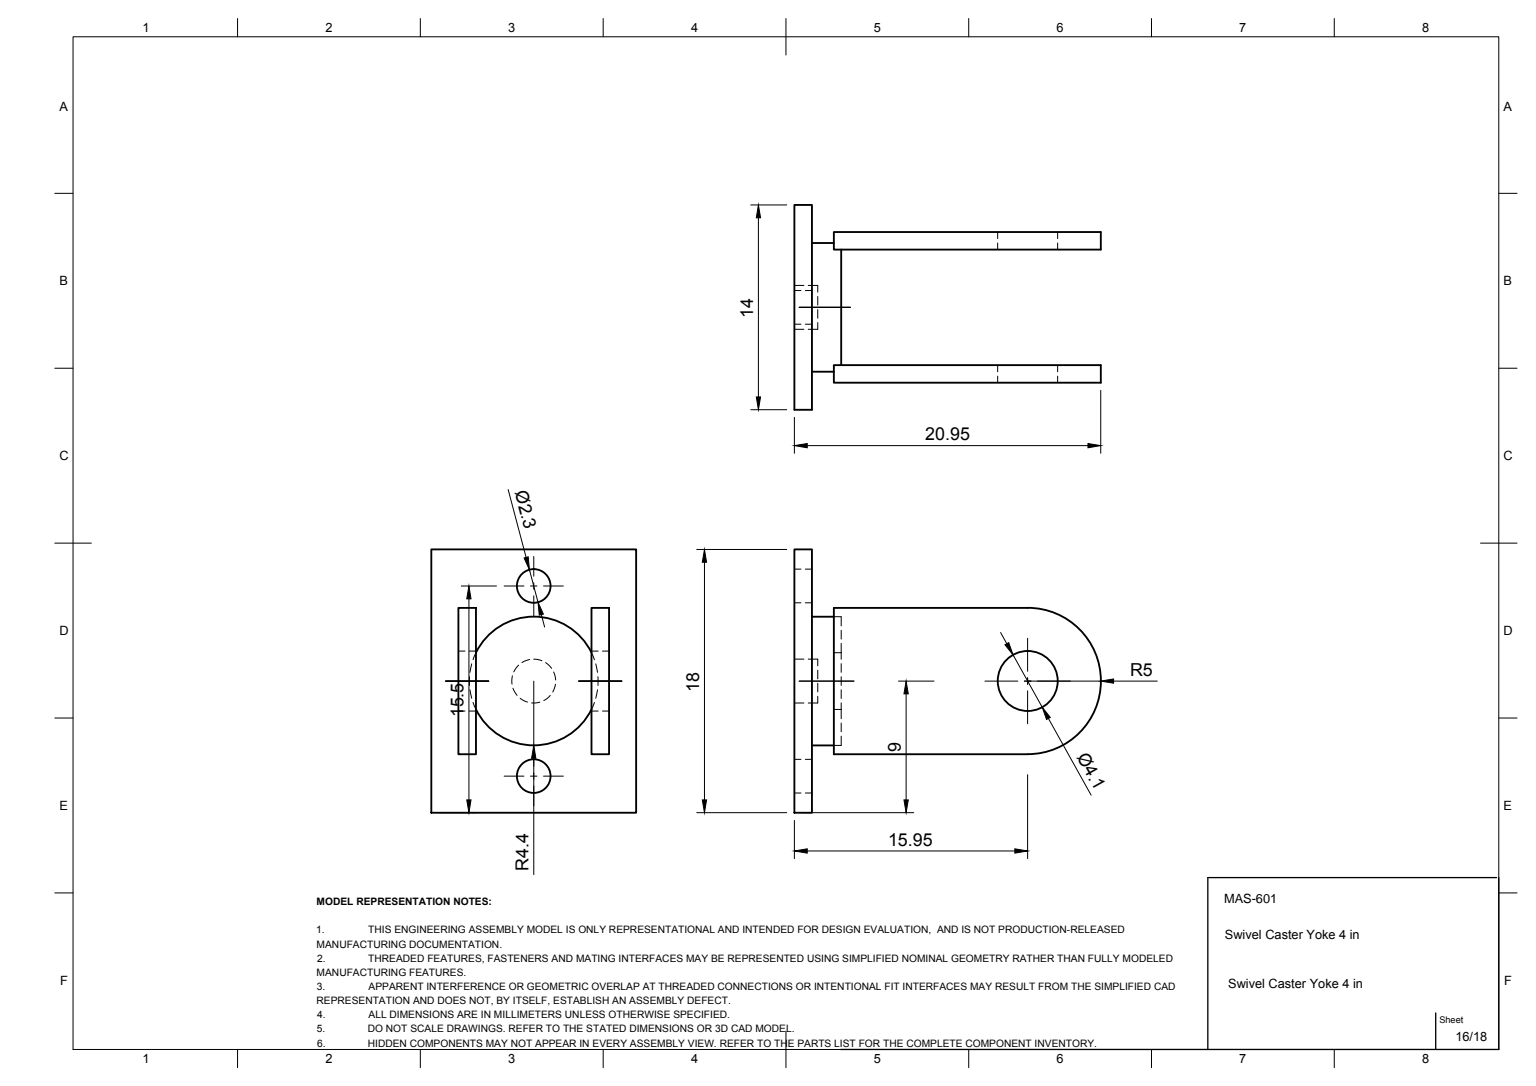
ISO-10303-21;
HEADER;
FILE_DESCRIPTION((''),'2;1');
FILE_NAME('Swivel Caster Yoke 4 in.step','2026-10-06T07:37:42+05:00',(''),(''),'','','');
FILE_SCHEMA (('AUTOMOTIVE_DESIGN { 1 0 10303 214 3 1 1 }'));
ENDSEC;
DATA;
#10=MECHANICAL_DESIGN_GEOMETRIC_PRESENTATION_REPRESENTATION('',(#387),#18757);
#353=SHAPE_REPRESENTATION_RELATIONSHIP('SRR','None',#18871,#370) ;
#370=ADVANCED_BREP_SHAPE_REPRESENTATION('',(#404),#18754) ;
#387=STYLED_ITEM('',(#18965),#404) ;
#404=MANIFOLD_SOLID_BREP('Swivel Caster Yoke 4 in',#9556) ;
#633=CYLINDRICAL_SURFACE('',#10553,1.15) ;
#634=CYLINDRICAL_SURFACE('',#10556,1.15) ;
#635=CYLINDRICAL_SURFACE('',#10561,2.04999999999999) ;
#636=CYLINDRICAL_SURFACE('',#10565,5.) ;
#637=CYLINDRICAL_SURFACE('',#10578,2.04999999999999) ;
#638=CYLINDRICAL_SURFACE('',#10581,5.) ;
#639=CYLINDRICAL_SURFACE('',#10587,4.4) ;
#640=CYLINDRICAL_SURFACE('',#10591,1.49999999999999) ;
#735=FACE_BOUND('',#2159,.T.) ;
#736=FACE_BOUND('',#2161,.T.) ;
#737=FACE_BOUND('',#2164,.T.) ;
#738=FACE_BOUND('',#2171,.T.) ;
#739=FACE_BOUND('',#2180,.T.) ;
#740=FACE_BOUND('',#2181,.T.) ;
#741=FACE_BOUND('',#2182,.T.) ;
#742=FACE_BOUND('',#2184,.T.) ;
#743=FACE_BOUND('',#2185,.T.) ;
#744=FACE_BOUND('',#2186,.T.) ;
#1051=PLANE('',#10559) ;
#1052=PLANE('',#10564) ;
#1053=PLANE('',#10568) ;
#1054=PLANE('',#10569) ;
#1055=PLANE('',#10570) ;
#1056=PLANE('',#10571) ;
#1057=PLANE('',#10575) ;
#1058=PLANE('',#10580) ;
#1059=PLANE('',#10583) ;
#1060=PLANE('',#10584) ;
#1061=PLANE('',#10586) ;
#1062=PLANE('',#10589) ;
#1063=PLANE('',#10593) ;
#1064=PLANE('',#10594) ;
#1065=PLANE('',#10595) ;
#1066=PLANE('',#10596) ;
#1067=PLANE('',#10597) ;
#1068=PLANE('',#10598) ;
#1548=FACE_OUTER_BOUND('',#2151,.T.) ;
#1549=FACE_OUTER_BOUND('',#2152,.T.) ;
#1550=FACE_OUTER_BOUND('',#2153,.T.) ;
#1551=FACE_OUTER_BOUND('',#2154,.T.) ;
#1552=FACE_OUTER_BOUND('',#2155,.T.) ;
#1553=FACE_OUTER_BOUND('',#2156,.T.) ;
#1554=FACE_OUTER_BOUND('',#2157,.T.) ;
#1555=FACE_OUTER_BOUND('',#2158,.T.) ;
#1556=FACE_OUTER_BOUND('',#2160,.T.) ;
#1557=FACE_OUTER_BOUND('',#2162,.T.) ;
#1558=FACE_OUTER_BOUND('',#2163,.T.) ;
#1559=FACE_OUTER_BOUND('',#2165,.T.) ;
#1560=FACE_OUTER_BOUND('',#2166,.T.) ;
#1561=FACE_OUTER_BOUND('',#2167,.T.) ;
#1562=FACE_OUTER_BOUND('',#2168,.T.) ;
#1563=FACE_OUTER_BOUND('',#2169,.T.) ;
#1564=FACE_OUTER_BOUND('',#2170,.T.) ;
#1565=FACE_OUTER_BOUND('',#2172,.T.) ;
#1566=FACE_OUTER_BOUND('',#2173,.T.) ;
#1567=FACE_OUTER_BOUND('',#2174,.T.) ;
#1568=FACE_OUTER_BOUND('',#2175,.T.) ;
#1569=FACE_OUTER_BOUND('',#2176,.T.) ;
#1570=FACE_OUTER_BOUND('',#2177,.T.) ;
#1571=FACE_OUTER_BOUND('',#2178,.T.) ;
#1572=FACE_OUTER_BOUND('',#2179,.T.) ;
#1573=FACE_OUTER_BOUND('',#2183,.T.) ;
#2151=EDGE_LOOP('',(#8725,#8726,#8727,#8728)) ;
#2152=EDGE_LOOP('',(#8729,#8730,#8731,#8732)) ;
#2153=EDGE_LOOP('',(#8733,#8734,#8735,#8736,#8737,#8738)) ;
#2154=EDGE_LOOP('',(#8739,#8740,#8741,#8742)) ;
#2155=EDGE_LOOP('',(#8743,#8744,#8745,#8746)) ;
#2156=EDGE_LOOP('',(#8747,#8748,#8749,#8750)) ;
#2157=EDGE_LOOP('',(#8751,#8752,#8753,#8754)) ;
#2158=EDGE_LOOP('',(#8755,#8756,#8757,#8758,#8759,#8760,#8761,#8762)) ;
#2159=EDGE_LOOP('',(#8763)) ;
#2160=EDGE_LOOP('',(#8764,#8765,#8766,#8767)) ;
#2161=EDGE_LOOP('',(#8768)) ;
#2162=EDGE_LOOP('',(#8769,#8770,#8771,#8772,#8773)) ;
#2163=EDGE_LOOP('',(#8774,#8775,#8776,#8777,#8778,#8779,#8780,#8781)) ;
#2164=EDGE_LOOP('',(#8782)) ;
#2165=EDGE_LOOP('',(#8783,#8784,#8785,#8786)) ;
#2166=EDGE_LOOP('',(#8787,#8788,#8789,#8790)) ;
#2167=EDGE_LOOP('',(#8791,#8792,#8793,#8794)) ;
#2168=EDGE_LOOP('',(#8795,#8796,#8797,#8798)) ;
#2169=EDGE_LOOP('',(#8799,#8800,#8801,#8802,#8803,#8804)) ;
#2170=EDGE_LOOP('',(#8805,#8806,#8807,#8808)) ;
#2171=EDGE_LOOP('',(#8809)) ;
#2172=EDGE_LOOP('',(#8810,#8811,#8812,#8813,#8814,#8815,#8816,#8817,#8818,
#8819,#8820,#8821)) ;
#2173=EDGE_LOOP('',(#8822)) ;
#2174=EDGE_LOOP('',(#8823,#8824,#8825,#8826)) ;
#2175=EDGE_LOOP('',(#8827,#8828,#8829,#8830)) ;
#2176=EDGE_LOOP('',(#8831,#8832,#8833,#8834)) ;
#2177=EDGE_LOOP('',(#8835,#8836,#8837,#8838)) ;
#2178=EDGE_LOOP('',(#8839,#8840,#8841,#8842)) ;
#2179=EDGE_LOOP('',(#8843,#8844,#8845,#8846)) ;
#2180=EDGE_LOOP('',(#8847)) ;
#2181=EDGE_LOOP('',(#8848)) ;
#2182=EDGE_LOOP('',(#8849)) ;
#2183=EDGE_LOOP('',(#8850,#8851,#8852,#8853)) ;
#2184=EDGE_LOOP('',(#8854)) ;
#2185=EDGE_LOOP('',(#8855)) ;
#2186=EDGE_LOOP('',(#8856)) ;
#2914=LINE('',#18384,#3685) ;
#2915=LINE('',#18390,#3686) ;
#2916=LINE('',#18397,#3687) ;
#2917=LINE('',#18399,#3688) ;
#2918=LINE('',#18401,#3689) ;
#2919=LINE('',#18403,#3690) ;
#2920=LINE('',#18404,#3691) ;
#2921=LINE('',#18409,#3692) ;
#2922=LINE('',#18413,#3693) ;
#2923=LINE('',#18415,#3694) ;
#2924=LINE('',#18416,#3695) ;
#2925=LINE('',#18422,#3696) ;
#2926=LINE('',#18424,#3697) ;
#2927=LINE('',#18425,#3698) ;
#2928=LINE('',#18428,#3699) ;
#2929=LINE('',#18430,#3700) ;
#2930=LINE('',#18431,#3701) ;
#2931=LINE('',#18439,#3702) ;
#2932=LINE('',#18443,#3703) ;
#2933=LINE('',#18445,#3704) ;
#2934=LINE('',#18447,#3705) ;
#2935=LINE('',#18449,#3706) ;
#2936=LINE('',#18453,#3707) ;
#2937=LINE('',#18454,#3708) ;
#2938=LINE('',#18460,#3709) ;
#2939=LINE('',#18463,#3710) ;
#2940=LINE('',#18465,#3711) ;
#2941=LINE('',#18466,#3712) ;
#2942=LINE('',#18470,#3713) ;
#2943=LINE('',#18473,#3714) ;
#2944=LINE('',#18474,#3715) ;
#2945=LINE('',#18477,#3716) ;
#2946=LINE('',#18482,#3717) ;
#2947=LINE('',#18488,#3718) ;
#2948=LINE('',#18493,#3719) ;
#2949=LINE('',#18495,#3720) ;
#2950=LINE('',#18497,#3721) ;
#2951=LINE('',#18498,#3722) ;
#2952=LINE('',#18501,#3723) ;
#2953=LINE('',#18503,#3724) ;
#2954=LINE('',#18504,#3725) ;
#2955=LINE('',#18507,#3726) ;
#2956=LINE('',#18509,#3727) ;
#2957=LINE('',#18510,#3728) ;
#2958=LINE('',#18512,#3729) ;
#2959=LINE('',#18513,#3730) ;
#3685=VECTOR('',#13012,1.15) ;
#3686=VECTOR('',#13019,1.15) ;
#3687=VECTOR('',#13026,10.) ;
#3688=VECTOR('',#13027,10.) ;
#3689=VECTOR('',#13028,10.) ;
#3690=VECTOR('',#13029,10.) ;
#3691=VECTOR('',#13030,10.) ;
#3692=VECTOR('',#13035,2.04999999999999) ;
#3693=VECTOR('',#13040,10.) ;
#3694=VECTOR('',#13041,10.) ;
#3695=VECTOR('',#13042,10.) ;
#3696=VECTOR('',#13049,10.) ;
#3697=VECTOR('',#13052,10.) ;
#3698=VECTOR('',#13053,10.) ;
#3699=VECTOR('',#13056,10.) ;
#3700=VECTOR('',#13057,10.) ;
#3701=VECTOR('',#13058,10.) ;
#3702=VECTOR('',#13067,10.) ;
#3703=VECTOR('',#13072,10.) ;
#3704=VECTOR('',#13073,10.) ;
#3705=VECTOR('',#13074,10.) ;
#3706=VECTOR('',#13075,10.) ;
#3707=VECTOR('',#13078,10.) ;
#3708=VECTOR('',#13079,10.) ;
#3709=VECTOR('',#13086,2.04999999999999) ;
#3710=VECTOR('',#13089,10.) ;
#3711=VECTOR('',#13090,10.) ;
#3712=VECTOR('',#13091,10.) ;
#3713=VECTOR('',#13096,10.) ;
#3714=VECTOR('',#13099,10.) ;
#3715=VECTOR('',#13100,10.) ;
#3716=VECTOR('',#13105,10.) ;
#3717=VECTOR('',#13112,4.4) ;
#3718=VECTOR('',#13119,1.49999999999999) ;
#3719=VECTOR('',#13124,10.) ;
#3720=VECTOR('',#13125,10.) ;
#3721=VECTOR('',#13126,10.) ;
#3722=VECTOR('',#13127,10.) ;
#3723=VECTOR('',#13130,10.) ;
#3724=VECTOR('',#13131,10.) ;
#3725=VECTOR('',#13132,10.) ;
#3726=VECTOR('',#13135,10.) ;
#3727=VECTOR('',#13136,10.) ;
#3728=VECTOR('',#13137,10.) ;
#3729=VECTOR('',#13140,10.) ;
#3730=VECTOR('',#13141,10.) ;
#4106=CIRCLE('',#10554,1.15) ;
#4107=CIRCLE('',#10555,1.15) ;
#4108=CIRCLE('',#10557,1.15) ;
#4109=CIRCLE('',#10558,1.15) ;
#4110=CIRCLE('',#10560,4.4) ;
#4111=CIRCLE('',#10562,2.04999999999999) ;
#4112=CIRCLE('',#10563,2.04999999999999) ;
#4113=CIRCLE('',#10566,5.) ;
#4114=CIRCLE('',#10567,5.) ;
#4115=CIRCLE('',#10572,4.4) ;
#4116=CIRCLE('',#10573,4.4) ;
#4117=CIRCLE('',#10574,4.4) ;
#4118=CIRCLE('',#10576,5.) ;
#4119=CIRCLE('',#10577,2.04999999999999) ;
#4120=CIRCLE('',#10579,2.04999999999999) ;
#4121=CIRCLE('',#10582,5.) ;
#4122=CIRCLE('',#10585,4.4) ;
#4123=CIRCLE('',#10588,4.4) ;
#4124=CIRCLE('',#10590,1.49999999999999) ;
#4125=CIRCLE('',#10592,1.49999999999999) ;
#4930=VERTEX_POINT('',#18381) ;
#4931=VERTEX_POINT('',#18383) ;
#4932=VERTEX_POINT('',#18387) ;
#4933=VERTEX_POINT('',#18389) ;
#4934=VERTEX_POINT('',#18393) ;
#4935=VERTEX_POINT('',#18394) ;
#4936=VERTEX_POINT('',#18396) ;
#4937=VERTEX_POINT('',#18398) ;
#4938=VERTEX_POINT('',#18400) ;
#4939=VERTEX_POINT('',#18402) ;
#4940=VERTEX_POINT('',#18406) ;
#4941=VERTEX_POINT('',#18408) ;
#4942=VERTEX_POINT('',#18412) ;
#4943=VERTEX_POINT('',#18414) ;
#4944=VERTEX_POINT('',#18418) ;
#4945=VERTEX_POINT('',#18420) ;
#4946=VERTEX_POINT('',#18427) ;
#4947=VERTEX_POINT('',#18429) ;
#4948=VERTEX_POINT('',#18434) ;
#4949=VERTEX_POINT('',#18436) ;
#4950=VERTEX_POINT('',#18438) ;
#4951=VERTEX_POINT('',#18442) ;
#4952=VERTEX_POINT('',#18444) ;
#4953=VERTEX_POINT('',#18446) ;
#4954=VERTEX_POINT('',#18448) ;
#4955=VERTEX_POINT('',#18450) ;
#4956=VERTEX_POINT('',#18452) ;
#4957=VERTEX_POINT('',#18455) ;
#4958=VERTEX_POINT('',#18458) ;
#4959=VERTEX_POINT('',#18462) ;
#4960=VERTEX_POINT('',#18464) ;
#4961=VERTEX_POINT('',#18468) ;
#4962=VERTEX_POINT('',#18472) ;
#4963=VERTEX_POINT('',#18480) ;
#4964=VERTEX_POINT('',#18484) ;
#4965=VERTEX_POINT('',#18487) ;
#4966=VERTEX_POINT('',#18491) ;
#4967=VERTEX_POINT('',#18492) ;
#4968=VERTEX_POINT('',#18494) ;
#4969=VERTEX_POINT('',#18496) ;
#4970=VERTEX_POINT('',#18500) ;
#4971=VERTEX_POINT('',#18502) ;
#4972=VERTEX_POINT('',#18506) ;
#4973=VERTEX_POINT('',#18508) ;
#6209=EDGE_CURVE('',#4930,#4930,#4106,.T.) ;
#6210=EDGE_CURVE('',#4930,#4931,#2914,.T.) ;
#6211=EDGE_CURVE('',#4931,#4931,#4107,.T.) ;
#6212=EDGE_CURVE('',#4932,#4932,#4108,.T.) ;
#6213=EDGE_CURVE('',#4932,#4933,#2915,.T.) ;
#6214=EDGE_CURVE('',#4933,#4933,#4109,.T.) ;
#6215=EDGE_CURVE('',#4934,#4935,#4110,.T.) ;
#6216=EDGE_CURVE('',#4936,#4934,#2916,.T.) ;
#6217=EDGE_CURVE('',#4937,#4936,#2917,.T.) ;
#6218=EDGE_CURVE('',#4937,#4938,#2918,.T.) ;
#6219=EDGE_CURVE('',#4938,#4939,#2919,.T.) ;
#6220=EDGE_CURVE('',#4935,#4939,#2920,.T.) ;
#6221=EDGE_CURVE('',#4940,#4940,#4111,.T.) ;
#6222=EDGE_CURVE('',#4940,#4941,#2921,.T.) ;
#6223=EDGE_CURVE('',#4941,#4941,#4112,.T.) ;
#6224=EDGE_CURVE('',#4942,#4937,#2922,.T.) ;
#6225=EDGE_CURVE('',#4943,#4936,#2923,.T.) ;
#6226=EDGE_CURVE('',#4942,#4943,#2924,.T.) ;
#6227=EDGE_CURVE('',#4944,#4942,#4113,.T.) ;
#6228=EDGE_CURVE('',#4945,#4943,#4114,.T.) ;
#6229=EDGE_CURVE('',#4944,#4945,#2925,.T.) ;
#6230=EDGE_CURVE('',#4938,#4944,#2926,.T.) ;
#6231=EDGE_CURVE('',#4939,#4945,#2927,.T.) ;
#6232=EDGE_CURVE('',#4935,#4946,#2928,.T.) ;
#6233=EDGE_CURVE('',#4947,#4934,#2929,.T.) ;
#6234=EDGE_CURVE('',#4946,#4947,#2930,.T.) ;
#6235=EDGE_CURVE('',#4948,#4947,#4115,.T.) ;
#6236=EDGE_CURVE('',#4949,#4948,#4116,.T.) ;
#6237=EDGE_CURVE('',#4949,#4950,#2931,.T.) ;
#6238=EDGE_CURVE('',#4946,#4950,#4117,.T.) ;
#6239=EDGE_CURVE('',#4950,#4951,#2932,.T.) ;
#6240=EDGE_CURVE('',#4952,#4949,#2933,.T.) ;
#6241=EDGE_CURVE('',#4953,#4952,#2934,.T.) ;
#6242=EDGE_CURVE('',#4954,#4953,#2935,.T.) ;
#6243=EDGE_CURVE('',#4955,#4954,#4118,.T.) ;
#6244=EDGE_CURVE('',#4956,#4955,#2936,.T.) ;
#6245=EDGE_CURVE('',#4951,#4956,#2937,.T.) ;
#6246=EDGE_CURVE('',#4957,#4957,#4119,.T.) ;
#6247=EDGE_CURVE('',#4958,#4958,#4120,.T.) ;
#6248=EDGE_CURVE('',#4958,#4957,#2938,.T.) ;
#6249=EDGE_CURVE('',#4953,#4959,#2939,.T.) ;
#6250=EDGE_CURVE('',#4960,#4959,#2940,.T.) ;
#6251=EDGE_CURVE('',#4954,#4960,#2941,.T.) ;
#6252=EDGE_CURVE('',#4961,#4960,#4121,.T.) ;
#6253=EDGE_CURVE('',#4955,#4961,#2942,.T.) ;
#6254=EDGE_CURVE('',#4962,#4961,#2943,.T.) ;
#6255=EDGE_CURVE('',#4956,#4962,#2944,.T.) ;
#6256=EDGE_CURVE('',#4951,#4952,#4122,.T.) ;
#6257=EDGE_CURVE('',#4959,#4962,#2945,.T.) ;
#6258=EDGE_CURVE('',#4963,#4963,#4123,.T.) ;
#6259=EDGE_CURVE('',#4963,#4948,#2946,.T.) ;
#6260=EDGE_CURVE('',#4964,#4964,#4124,.T.) ;
#6261=EDGE_CURVE('',#4964,#4965,#2947,.T.) ;
#6262=EDGE_CURVE('',#4965,#4965,#4125,.T.) ;
#6263=EDGE_CURVE('',#4966,#4967,#2948,.T.) ;
#6264=EDGE_CURVE('',#4967,#4968,#2949,.T.) ;
#6265=EDGE_CURVE('',#4969,#4968,#2950,.T.) ;
#6266=EDGE_CURVE('',#4966,#4969,#2951,.T.) ;
#6267=EDGE_CURVE('',#4970,#4966,#2952,.T.) ;
#6268=EDGE_CURVE('',#4971,#4969,#2953,.T.) ;
#6269=EDGE_CURVE('',#4970,#4971,#2954,.T.) ;
#6270=EDGE_CURVE('',#4972,#4970,#2955,.T.) ;
#6271=EDGE_CURVE('',#4973,#4971,#2956,.T.) ;
#6272=EDGE_CURVE('',#4972,#4973,#2957,.T.) ;
#6273=EDGE_CURVE('',#4967,#4972,#2958,.T.) ;
#6274=EDGE_CURVE('',#4968,#4973,#2959,.T.) ;
#8725=ORIENTED_EDGE('',*,*,#6209,.F.) ;
#8726=ORIENTED_EDGE('',*,*,#6210,.T.) ;
#8727=ORIENTED_EDGE('',*,*,#6211,.F.) ;
#8728=ORIENTED_EDGE('',*,*,#6210,.F.) ;
#8729=ORIENTED_EDGE('',*,*,#6212,.F.) ;
#8730=ORIENTED_EDGE('',*,*,#6213,.T.) ;
#8731=ORIENTED_EDGE('',*,*,#6214,.F.) ;
#8732=ORIENTED_EDGE('',*,*,#6213,.F.) ;
#8733=ORIENTED_EDGE('',*,*,#6215,.F.) ;
#8734=ORIENTED_EDGE('',*,*,#6216,.F.) ;
#8735=ORIENTED_EDGE('',*,*,#6217,.F.) ;
#8736=ORIENTED_EDGE('',*,*,#6218,.T.) ;
#8737=ORIENTED_EDGE('',*,*,#6219,.T.) ;
#8738=ORIENTED_EDGE('',*,*,#6220,.F.) ;
#8739=ORIENTED_EDGE('',*,*,#6221,.F.) ;
#8740=ORIENTED_EDGE('',*,*,#6222,.T.) ;
#8741=ORIENTED_EDGE('',*,*,#6223,.T.) ;
#8742=ORIENTED_EDGE('',*,*,#6222,.F.) ;
#8743=ORIENTED_EDGE('',*,*,#6224,.T.) ;
#8744=ORIENTED_EDGE('',*,*,#6217,.T.) ;
#8745=ORIENTED_EDGE('',*,*,#6225,.F.) ;
#8746=ORIENTED_EDGE('',*,*,#6226,.F.) ;
#8747=ORIENTED_EDGE('',*,*,#6227,.T.) ;
#8748=ORIENTED_EDGE('',*,*,#6226,.T.) ;
#8749=ORIENTED_EDGE('',*,*,#6228,.F.) ;
#8750=ORIENTED_EDGE('',*,*,#6229,.F.) ;
#8751=ORIENTED_EDGE('',*,*,#6230,.T.) ;
#8752=ORIENTED_EDGE('',*,*,#6229,.T.) ;
#8753=ORIENTED_EDGE('',*,*,#6231,.F.) ;
#8754=ORIENTED_EDGE('',*,*,#6219,.F.) ;
#8755=ORIENTED_EDGE('',*,*,#6232,.F.) ;
#8756=ORIENTED_EDGE('',*,*,#6220,.T.) ;
#8757=ORIENTED_EDGE('',*,*,#6231,.T.) ;
#8758=ORIENTED_EDGE('',*,*,#6228,.T.) ;
#8759=ORIENTED_EDGE('',*,*,#6225,.T.) ;
#8760=ORIENTED_EDGE('',*,*,#6216,.T.) ;
#8761=ORIENTED_EDGE('',*,*,#6233,.F.) ;
#8762=ORIENTED_EDGE('',*,*,#6234,.F.) ;
#8763=ORIENTED_EDGE('',*,*,#6221,.T.) ;
#8764=ORIENTED_EDGE('',*,*,#6218,.F.) ;
#8765=ORIENTED_EDGE('',*,*,#6224,.F.) ;
#8766=ORIENTED_EDGE('',*,*,#6227,.F.) ;
#8767=ORIENTED_EDGE('',*,*,#6230,.F.) ;
#8768=ORIENTED_EDGE('',*,*,#6223,.F.) ;
#8769=ORIENTED_EDGE('',*,*,#6234,.T.) ;
#8770=ORIENTED_EDGE('',*,*,#6235,.F.) ;
#8771=ORIENTED_EDGE('',*,*,#6236,.F.) ;
#8772=ORIENTED_EDGE('',*,*,#6237,.T.) ;
#8773=ORIENTED_EDGE('',*,*,#6238,.F.) ;
#8774=ORIENTED_EDGE('',*,*,#6239,.F.) ;
#8775=ORIENTED_EDGE('',*,*,#6237,.F.) ;
#8776=ORIENTED_EDGE('',*,*,#6240,.F.) ;
#8777=ORIENTED_EDGE('',*,*,#6241,.F.) ;
#8778=ORIENTED_EDGE('',*,*,#6242,.F.) ;
#8779=ORIENTED_EDGE('',*,*,#6243,.F.) ;
#8780=ORIENTED_EDGE('',*,*,#6244,.F.) ;
#8781=ORIENTED_EDGE('',*,*,#6245,.F.) ;
#8782=ORIENTED_EDGE('',*,*,#6246,.F.) ;
#8783=ORIENTED_EDGE('',*,*,#6247,.F.) ;
#8784=ORIENTED_EDGE('',*,*,#6248,.T.) ;
#8785=ORIENTED_EDGE('',*,*,#6246,.T.) ;
#8786=ORIENTED_EDGE('',*,*,#6248,.F.) ;
#8787=ORIENTED_EDGE('',*,*,#6242,.T.) ;
#8788=ORIENTED_EDGE('',*,*,#6249,.T.) ;
#8789=ORIENTED_EDGE('',*,*,#6250,.F.) ;
#8790=ORIENTED_EDGE('',*,*,#6251,.F.) ;
#8791=ORIENTED_EDGE('',*,*,#6243,.T.) ;
#8792=ORIENTED_EDGE('',*,*,#6251,.T.) ;
#8793=ORIENTED_EDGE('',*,*,#6252,.F.) ;
#8794=ORIENTED_EDGE('',*,*,#6253,.F.) ;
#8795=ORIENTED_EDGE('',*,*,#6244,.T.) ;
#8796=ORIENTED_EDGE('',*,*,#6253,.T.) ;
#8797=ORIENTED_EDGE('',*,*,#6254,.F.) ;
#8798=ORIENTED_EDGE('',*,*,#6255,.F.) ;
#8799=ORIENTED_EDGE('',*,*,#6256,.F.) ;
#8800=ORIENTED_EDGE('',*,*,#6245,.T.) ;
#8801=ORIENTED_EDGE('',*,*,#6255,.T.) ;
#8802=ORIENTED_EDGE('',*,*,#6257,.F.) ;
#8803=ORIENTED_EDGE('',*,*,#6249,.F.) ;
#8804=ORIENTED_EDGE('',*,*,#6241,.T.) ;
#8805=ORIENTED_EDGE('',*,*,#6257,.T.) ;
#8806=ORIENTED_EDGE('',*,*,#6254,.T.) ;
#8807=ORIENTED_EDGE('',*,*,#6252,.T.) ;
#8808=ORIENTED_EDGE('',*,*,#6250,.T.) ;
#8809=ORIENTED_EDGE('',*,*,#6247,.T.) ;
#8810=ORIENTED_EDGE('',*,*,#6258,.F.) ;
#8811=ORIENTED_EDGE('',*,*,#6259,.T.) ;
#8812=ORIENTED_EDGE('',*,*,#6235,.T.) ;
#8813=ORIENTED_EDGE('',*,*,#6233,.T.) ;
#8814=ORIENTED_EDGE('',*,*,#6215,.T.) ;
#8815=ORIENTED_EDGE('',*,*,#6232,.T.) ;
#8816=ORIENTED_EDGE('',*,*,#6238,.T.) ;
#8817=ORIENTED_EDGE('',*,*,#6239,.T.) ;
#8818=ORIENTED_EDGE('',*,*,#6256,.T.) ;
#8819=ORIENTED_EDGE('',*,*,#6240,.T.) ;
#8820=ORIENTED_EDGE('',*,*,#6236,.T.) ;
#8821=ORIENTED_EDGE('',*,*,#6259,.F.) ;
#8822=ORIENTED_EDGE('',*,*,#6260,.T.) ;
#8823=ORIENTED_EDGE('',*,*,#6260,.F.) ;
#8824=ORIENTED_EDGE('',*,*,#6261,.T.) ;
#8825=ORIENTED_EDGE('',*,*,#6262,.F.) ;
#8826=ORIENTED_EDGE('',*,*,#6261,.F.) ;
#8827=ORIENTED_EDGE('',*,*,#6263,.T.) ;
#8828=ORIENTED_EDGE('',*,*,#6264,.T.) ;
#8829=ORIENTED_EDGE('',*,*,#6265,.F.) ;
#8830=ORIENTED_EDGE('',*,*,#6266,.F.) ;
#8831=ORIENTED_EDGE('',*,*,#6267,.T.) ;
#8832=ORIENTED_EDGE('',*,*,#6266,.T.) ;
#8833=ORIENTED_EDGE('',*,*,#6268,.F.) ;
#8834=ORIENTED_EDGE('',*,*,#6269,.F.) ;
#8835=ORIENTED_EDGE('',*,*,#6270,.T.) ;
#8836=ORIENTED_EDGE('',*,*,#6269,.T.) ;
#8837=ORIENTED_EDGE('',*,*,#6271,.F.) ;
#8838=ORIENTED_EDGE('',*,*,#6272,.F.) ;
#8839=ORIENTED_EDGE('',*,*,#6273,.T.) ;
#8840=ORIENTED_EDGE('',*,*,#6272,.T.) ;
#8841=ORIENTED_EDGE('',*,*,#6274,.F.) ;
#8842=ORIENTED_EDGE('',*,*,#6264,.F.) ;
#8843=ORIENTED_EDGE('',*,*,#6274,.T.) ;
#8844=ORIENTED_EDGE('',*,*,#6271,.T.) ;
#8845=ORIENTED_EDGE('',*,*,#6268,.T.) ;
#8846=ORIENTED_EDGE('',*,*,#6265,.T.) ;
#8847=ORIENTED_EDGE('',*,*,#6209,.T.) ;
#8848=ORIENTED_EDGE('',*,*,#6212,.T.) ;
#8849=ORIENTED_EDGE('',*,*,#6262,.T.) ;
#8850=ORIENTED_EDGE('',*,*,#6273,.F.) ;
#8851=ORIENTED_EDGE('',*,*,#6263,.F.) ;
#8852=ORIENTED_EDGE('',*,*,#6267,.F.) ;
#8853=ORIENTED_EDGE('',*,*,#6270,.F.) ;
#8854=ORIENTED_EDGE('',*,*,#6211,.T.) ;
#8855=ORIENTED_EDGE('',*,*,#6214,.T.) ;
#8856=ORIENTED_EDGE('',*,*,#6258,.T.) ;
#9484=ADVANCED_FACE('',(#1548),#633,.F.) ;
#9485=ADVANCED_FACE('',(#1549),#634,.F.) ;
#9486=ADVANCED_FACE('',(#1550),#1051,.T.) ;
#9487=ADVANCED_FACE('',(#1551),#635,.F.) ;
#9488=ADVANCED_FACE('',(#1552),#1052,.T.) ;
#9489=ADVANCED_FACE('',(#1553),#636,.T.) ;
#9490=ADVANCED_FACE('',(#1554),#1053,.T.) ;
#9491=ADVANCED_FACE('',(#1555,#735),#1054,.T.) ;
#9492=ADVANCED_FACE('',(#1556,#736),#1055,.F.) ;
#9493=ADVANCED_FACE('',(#1557),#1056,.T.) ;
#9494=ADVANCED_FACE('',(#1558,#737),#1057,.F.) ;
#9495=ADVANCED_FACE('',(#1559),#637,.F.) ;
#9496=ADVANCED_FACE('',(#1560),#1058,.T.) ;
#9497=ADVANCED_FACE('',(#1561),#638,.T.) ;
#9498=ADVANCED_FACE('',(#1562),#1059,.T.) ;
#9499=ADVANCED_FACE('',(#1563),#1060,.T.) ;
#9500=ADVANCED_FACE('',(#1564,#738),#1061,.T.) ;
#9501=ADVANCED_FACE('',(#1565),#639,.T.) ;
#9502=ADVANCED_FACE('',(#1566),#1062,.F.) ;
#9503=ADVANCED_FACE('',(#1567),#640,.F.) ;
#9504=ADVANCED_FACE('',(#1568),#1063,.T.) ;
#9505=ADVANCED_FACE('',(#1569),#1064,.T.) ;
#9506=ADVANCED_FACE('',(#1570),#1065,.T.) ;
#9507=ADVANCED_FACE('',(#1571),#1066,.T.) ;
#9508=ADVANCED_FACE('',(#1572,#739,#740,#741),#1067,.T.) ;
#9509=ADVANCED_FACE('',(#1573,#742,#743,#744),#1068,.F.) ;
#9556=CLOSED_SHELL('',(#9484,#9485,#9486,#9487,#9488,#9489,#9490,#9491,
#9492,#9493,#9494,#9495,#9496,#9497,#9498,#9499,#9500,#9501,#9502,#9503,
#9504,#9505,#9506,#9507,#9508,#9509)) ;
#10552=AXIS2_PLACEMENT_3D('',#18379,#13006,#13007) ;
#10553=AXIS2_PLACEMENT_3D('',#18380,#13008,#13009) ;
#10554=AXIS2_PLACEMENT_3D('',#18382,#13010,#13011) ;
#10555=AXIS2_PLACEMENT_3D('',#18385,#13013,#13014) ;
#10556=AXIS2_PLACEMENT_3D('',#18386,#13015,#13016) ;
#10557=AXIS2_PLACEMENT_3D('',#18388,#13017,#13018) ;
#10558=AXIS2_PLACEMENT_3D('',#18391,#13020,#13021) ;
#10559=AXIS2_PLACEMENT_3D('',#18392,#13022,#13023) ;
#10560=AXIS2_PLACEMENT_3D('',#18395,#13024,#13025) ;
#10561=AXIS2_PLACEMENT_3D('',#18405,#13031,#13032) ;
#10562=AXIS2_PLACEMENT_3D('',#18407,#13033,#13034) ;
#10563=AXIS2_PLACEMENT_3D('',#18410,#13036,#13037) ;
#10564=AXIS2_PLACEMENT_3D('',#18411,#13038,#13039) ;
#10565=AXIS2_PLACEMENT_3D('',#18417,#13043,#13044) ;
#10566=AXIS2_PLACEMENT_3D('',#18419,#13045,#13046) ;
#10567=AXIS2_PLACEMENT_3D('',#18421,#13047,#13048) ;
#10568=AXIS2_PLACEMENT_3D('',#18423,#13050,#13051) ;
#10569=AXIS2_PLACEMENT_3D('',#18426,#13054,#13055) ;
#10570=AXIS2_PLACEMENT_3D('',#18432,#13059,#13060) ;
#10571=AXIS2_PLACEMENT_3D('',#18433,#13061,#13062) ;
#10572=AXIS2_PLACEMENT_3D('',#18435,#13063,#13064) ;
#10573=AXIS2_PLACEMENT_3D('',#18437,#13065,#13066) ;
#10574=AXIS2_PLACEMENT_3D('',#18440,#13068,#13069) ;
#10575=AXIS2_PLACEMENT_3D('',#18441,#13070,#13071) ;
#10576=AXIS2_PLACEMENT_3D('',#18451,#13076,#13077) ;
#10577=AXIS2_PLACEMENT_3D('',#18456,#13080,#13081) ;
#10578=AXIS2_PLACEMENT_3D('',#18457,#13082,#13083) ;
#10579=AXIS2_PLACEMENT_3D('',#18459,#13084,#13085) ;
#10580=AXIS2_PLACEMENT_3D('',#18461,#13087,#13088) ;
#10581=AXIS2_PLACEMENT_3D('',#18467,#13092,#13093) ;
#10582=AXIS2_PLACEMENT_3D('',#18469,#13094,#13095) ;
#10583=AXIS2_PLACEMENT_3D('',#18471,#13097,#13098) ;
#10584=AXIS2_PLACEMENT_3D('',#18475,#13101,#13102) ;
#10585=AXIS2_PLACEMENT_3D('',#18476,#13103,#13104) ;
#10586=AXIS2_PLACEMENT_3D('',#18478,#13106,#13107) ;
#10587=AXIS2_PLACEMENT_3D('',#18479,#13108,#13109) ;
#10588=AXIS2_PLACEMENT_3D('',#18481,#13110,#13111) ;
#10589=AXIS2_PLACEMENT_3D('',#18483,#13113,#13114) ;
#10590=AXIS2_PLACEMENT_3D('',#18485,#13115,#13116) ;
#10591=AXIS2_PLACEMENT_3D('',#18486,#13117,#13118) ;
#10592=AXIS2_PLACEMENT_3D('',#18489,#13120,#13121) ;
#10593=AXIS2_PLACEMENT_3D('',#18490,#13122,#13123) ;
#10594=AXIS2_PLACEMENT_3D('',#18499,#13128,#13129) ;
#10595=AXIS2_PLACEMENT_3D('',#18505,#13133,#13134) ;
#10596=AXIS2_PLACEMENT_3D('',#18511,#13138,#13139) ;
#10597=AXIS2_PLACEMENT_3D('',#18514,#13142,#13143) ;
#10598=AXIS2_PLACEMENT_3D('',#18515,#13144,#13145) ;
#13006=DIRECTION('axis',(0.,0.,1.)) ;
#13007=DIRECTION('refdir',(1.,0.,0.)) ;
#13008=DIRECTION('center_axis',(0.,0.,-1.)) ;
#13009=DIRECTION('ref_axis',(1.,0.,0.)) ;
#13010=DIRECTION('center_axis',(0.,0.,-1.)) ;
#13011=DIRECTION('ref_axis',(1.,0.,0.)) ;
#13012=DIRECTION('',(0.,0.,-1.)) ;
#13013=DIRECTION('center_axis',(0.,0.,1.)) ;
#13014=DIRECTION('ref_axis',(1.,0.,0.)) ;
#13015=DIRECTION('center_axis',(0.,0.,-1.)) ;
#13016=DIRECTION('ref_axis',(1.,0.,0.)) ;
#13017=DIRECTION('center_axis',(0.,0.,-1.)) ;
#13018=DIRECTION('ref_axis',(1.,0.,0.)) ;
#13019=DIRECTION('',(0.,0.,-1.)) ;
#13020=DIRECTION('center_axis',(0.,0.,1.)) ;
#13021=DIRECTION('ref_axis',(1.,0.,0.)) ;
#13022=DIRECTION('center_axis',(0.,0.,1.)) ;
#13023=DIRECTION('ref_axis',(1.,0.,0.)) ;
#13024=DIRECTION('center_axis',(0.,0.,1.)) ;
#13025=DIRECTION('ref_axis',(1.,0.,0.)) ;
#13026=DIRECTION('',(1.,0.,0.)) ;
#13027=DIRECTION('',(0.,1.,0.)) ;
#13028=DIRECTION('',(1.,0.,0.)) ;
#13029=DIRECTION('',(0.,1.,0.)) ;
#13030=DIRECTION('',(1.,0.,0.)) ;
#13031=DIRECTION('center_axis',(0.,1.,0.)) ;
#13032=DIRECTION('ref_axis',(1.,0.,0.)) ;
#13033=DIRECTION('center_axis',(0.,-1.,0.)) ;
#13034=DIRECTION('ref_axis',(1.,0.,0.)) ;
#13035=DIRECTION('',(0.,-1.,0.)) ;
#13036=DIRECTION('center_axis',(0.,-1.,0.)) ;
#13037=DIRECTION('ref_axis',(1.,0.,0.)) ;
#13038=DIRECTION('center_axis',(-1.,0.,0.)) ;
#13039=DIRECTION('ref_axis',(0.,0.,1.)) ;
#13040=DIRECTION('',(0.,0.,1.)) ;
#13041=DIRECTION('',(0.,0.,1.)) ;
#13042=DIRECTION('',(0.,1.,0.)) ;
#13043=DIRECTION('center_axis',(0.,1.,0.)) ;
#13044=DIRECTION('ref_axis',(1.,0.,1.33226762955019E-15)) ;
#13045=DIRECTION('center_axis',(0.,1.,0.)) ;
#13046=DIRECTION('ref_axis',(1.,0.,1.33226762955019E-15)) ;
#13047=DIRECTION('center_axis',(0.,1.,0.)) ;
#13048=DIRECTION('ref_axis',(1.,0.,1.33226762955019E-15)) ;
#13049=DIRECTION('',(0.,1.,0.)) ;
#13050=DIRECTION('center_axis',(1.,0.,0.)) ;
#13051=DIRECTION('ref_axis',(0.,0.,-1.)) ;
#13052=DIRECTION('',(0.,0.,-1.)) ;
#13053=DIRECTION('',(0.,0.,-1.)) ;
#13054=DIRECTION('center_axis',(0.,1.,0.)) ;
#13055=DIRECTION('ref_axis',(1.,0.,0.)) ;
#13056=DIRECTION('',(0.,0.,-1.)) ;
#13057=DIRECTION('',(0.,0.,1.)) ;
#13058=DIRECTION('',(-1.,0.,0.)) ;
#13059=DIRECTION('center_axis',(0.,1.,0.)) ;
#13060=DIRECTION('ref_axis',(1.,0.,0.)) ;
#13061=DIRECTION('center_axis',(0.,0.,-1.)) ;
#13062=DIRECTION('ref_axis',(-1.,0.,0.)) ;
#13063=DIRECTION('center_axis',(0.,0.,1.)) ;
#13064=DIRECTION('ref_axis',(1.,0.,0.)) ;
#13065=DIRECTION('center_axis',(0.,0.,1.)) ;
#13066=DIRECTION('ref_axis',(1.,0.,0.)) ;
#13067=DIRECTION('',(1.,0.,0.)) ;
#13068=DIRECTION('center_axis',(0.,0.,1.)) ;
#13069=DIRECTION('ref_axis',(1.,0.,0.)) ;
#13070=DIRECTION('center_axis',(0.,1.,0.)) ;
#13071=DIRECTION('ref_axis',(1.,0.,0.)) ;
#13072=DIRECTION('',(0.,0.,1.)) ;
#13073=DIRECTION('',(0.,0.,-1.)) ;
#13074=DIRECTION('',(1.,0.,0.)) ;
#13075=DIRECTION('',(0.,0.,1.)) ;
#13076=DIRECTION('center_axis',(0.,1.,0.)) ;
#13077=DIRECTION('ref_axis',(1.,0.,1.33226762955019E-15)) ;
#13078=DIRECTION('',(0.,0.,-1.)) ;
#13079=DIRECTION('',(1.,0.,0.)) ;
#13080=DIRECTION('center_axis',(0.,-1.,0.)) ;
#13081=DIRECTION('ref_axis',(1.,0.,0.)) ;
#13082=DIRECTION('center_axis',(0.,1.,0.)) ;
#13083=DIRECTION('ref_axis',(1.,0.,0.)) ;
#13084=DIRECTION('center_axis',(0.,-1.,0.)) ;
#13085=DIRECTION('ref_axis',(1.,0.,0.)) ;
#13086=DIRECTION('',(0.,-1.,0.)) ;
#13087=DIRECTION('center_axis',(-1.,0.,0.)) ;
#13088=DIRECTION('ref_axis',(0.,0.,1.)) ;
#13089=DIRECTION('',(0.,1.,0.)) ;
#13090=DIRECTION('',(0.,0.,1.)) ;
#13091=DIRECTION('',(0.,1.,0.)) ;
#13092=DIRECTION('center_axis',(0.,1.,0.)) ;
#13093=DIRECTION('ref_axis',(1.,0.,1.33226762955019E-15)) ;
#13094=DIRECTION('center_axis',(0.,1.,0.)) ;
#13095=DIRECTION('ref_axis',(1.,0.,1.33226762955019E-15)) ;
#13096=DIRECTION('',(0.,1.,0.)) ;
#13097=DIRECTION('center_axis',(1.,0.,0.)) ;
#13098=DIRECTION('ref_axis',(0.,0.,-1.)) ;
#13099=DIRECTION('',(0.,0.,-1.)) ;
#13100=DIRECTION('',(0.,1.,0.)) ;
#13101=DIRECTION('center_axis',(0.,0.,1.)) ;
#13102=DIRECTION('ref_axis',(1.,0.,0.)) ;
#13103=DIRECTION('center_axis',(0.,0.,1.)) ;
#13104=DIRECTION('ref_axis',(1.,0.,0.)) ;
#13105=DIRECTION('',(1.,0.,0.)) ;
#13106=DIRECTION('center_axis',(0.,1.,0.)) ;
#13107=DIRECTION('ref_axis',(1.,0.,0.)) ;
#13108=DIRECTION('center_axis',(0.,0.,1.)) ;
#13109=DIRECTION('ref_axis',(1.,0.,0.)) ;
#13110=DIRECTION('center_axis',(0.,0.,1.)) ;
#13111=DIRECTION('ref_axis',(1.,0.,0.)) ;
#13112=DIRECTION('',(0.,0.,-1.)) ;
#13113=DIRECTION('center_axis',(0.,0.,-1.)) ;
#13114=DIRECTION('ref_axis',(-1.,0.,0.)) ;
#13115=DIRECTION('center_axis',(0.,0.,1.)) ;
#13116=DIRECTION('ref_axis',(1.,0.,0.)) ;
#13117=DIRECTION('center_axis',(0.,0.,1.)) ;
#13118=DIRECTION('ref_axis',(1.,0.,0.)) ;
#13119=DIRECTION('',(0.,0.,1.)) ;
#13120=DIRECTION('center_axis',(0.,0.,-1.)) ;
#13121=DIRECTION('ref_axis',(1.,0.,0.)) ;
#13122=DIRECTION('center_axis',(0.,1.,0.)) ;
#13123=DIRECTION('ref_axis',(-1.,0.,0.)) ;
#13124=DIRECTION('',(-1.,0.,0.)) ;
#13125=DIRECTION('',(0.,0.,1.)) ;
#13126=DIRECTION('',(-1.,0.,0.)) ;
#13127=DIRECTION('',(0.,0.,1.)) ;
#13128=DIRECTION('center_axis',(1.,0.,0.)) ;
#13129=DIRECTION('ref_axis',(0.,1.,0.)) ;
#13130=DIRECTION('',(0.,1.,0.)) ;
#13131=DIRECTION('',(0.,1.,0.)) ;
#13132=DIRECTION('',(0.,0.,1.)) ;
#13133=DIRECTION('center_axis',(0.,-1.,0.)) ;
#13134=DIRECTION('ref_axis',(1.,0.,0.)) ;
#13135=DIRECTION('',(1.,0.,0.)) ;
#13136=DIRECTION('',(1.,0.,0.)) ;
#13137=DIRECTION('',(0.,0.,1.)) ;
#13138=DIRECTION('center_axis',(-1.,0.,0.)) ;
#13139=DIRECTION('ref_axis',(0.,-1.,0.)) ;
#13140=DIRECTION('',(0.,-1.,0.)) ;
#13141=DIRECTION('',(0.,-1.,0.)) ;
#13142=DIRECTION('center_axis',(0.,0.,1.)) ;
#13143=DIRECTION('ref_axis',(1.,0.,0.)) ;
#13144=DIRECTION('center_axis',(0.,0.,1.)) ;
#13145=DIRECTION('ref_axis',(1.,0.,0.)) ;
#18379=CARTESIAN_POINT('',(0.,0.,0.)) ;
#18380=CARTESIAN_POINT('Origin',(84.75,52.3,27.6)) ;
#18381=CARTESIAN_POINT('',(83.6,52.3,27.6)) ;
#18382=CARTESIAN_POINT('Origin',(84.75,52.3,27.6)) ;
#18383=CARTESIAN_POINT('',(83.6,52.3,26.4)) ;
#18384=CARTESIAN_POINT('',(83.6,52.3,27.6)) ;
#18385=CARTESIAN_POINT('Origin',(84.75,52.3,26.4)) ;
#18386=CARTESIAN_POINT('Origin',(71.75,52.3,27.6)) ;
#18387=CARTESIAN_POINT('',(70.6,52.3,27.6)) ;
#18388=CARTESIAN_POINT('Origin',(71.75,52.3,27.6)) ;
#18389=CARTESIAN_POINT('',(70.6,52.3,26.4)) ;
#18390=CARTESIAN_POINT('',(70.6,52.3,27.6)) ;
#18391=CARTESIAN_POINT('Origin',(71.75,52.3,26.4)) ;
#18392=CARTESIAN_POINT('Origin',(73.25,47.15,24.9)) ;
#18393=CARTESIAN_POINT('',(76.311572802502,48.35,24.9)) ;
#18394=CARTESIAN_POINT('',(80.188427197498,48.35,24.9)) ;
#18395=CARTESIAN_POINT('Origin',(78.25,52.3,24.9)) ;
#18396=CARTESIAN_POINT('',(73.25,48.35,24.9)) ;
#18397=CARTESIAN_POINT('',(73.25,48.35,24.9)) ;
#18398=CARTESIAN_POINT('',(73.25,47.15,24.9)) ;
#18399=CARTESIAN_POINT('',(73.25,47.15,24.9)) ;
#18400=CARTESIAN_POINT('',(83.25,47.15,24.9)) ;
#18401=CARTESIAN_POINT('',(73.25,47.15,24.9)) ;
#18402=CARTESIAN_POINT('',(83.25,48.35,24.9)) ;
#18403=CARTESIAN_POINT('',(83.25,47.15,24.9)) ;
#18404=CARTESIAN_POINT('',(73.25,48.35,24.9)) ;
#18405=CARTESIAN_POINT('Origin',(78.25,47.15,11.65)) ;
#18406=CARTESIAN_POINT('',(76.2,48.35,11.65)) ;
#18407=CARTESIAN_POINT('Origin',(78.25,48.35,11.65)) ;
#18408=CARTESIAN_POINT('',(76.2,47.15,11.65)) ;
#18409=CARTESIAN_POINT('',(76.2,47.15,11.65)) ;
#18410=CARTESIAN_POINT('Origin',(78.25,47.15,11.65)) ;
#18411=CARTESIAN_POINT('Origin',(73.25,47.15,11.65)) ;
#18412=CARTESIAN_POINT('',(73.25,47.15,11.65)) ;
#18413=CARTESIAN_POINT('',(73.25,47.15,11.65)) ;
#18414=CARTESIAN_POINT('',(73.25,48.35,11.65)) ;
#18415=CARTESIAN_POINT('',(73.25,48.35,11.65)) ;
#18416=CARTESIAN_POINT('',(73.25,47.15,11.65)) ;
#18417=CARTESIAN_POINT('Origin',(78.25,47.15,11.65)) ;
#18418=CARTESIAN_POINT('',(83.25,47.15,11.65)) ;
#18419=CARTESIAN_POINT('Origin',(78.25,47.15,11.65)) ;
#18420=CARTESIAN_POINT('',(83.25,48.35,11.65)) ;
#18421=CARTESIAN_POINT('Origin',(78.25,48.35,11.65)) ;
#18422=CARTESIAN_POINT('',(83.25,47.15,11.65)) ;
#18423=CARTESIAN_POINT('Origin',(83.25,47.15,24.9)) ;
#18424=CARTESIAN_POINT('',(83.25,47.15,24.9)) ;
#18425=CARTESIAN_POINT('',(83.25,48.35,24.9)) ;
#18426=CARTESIAN_POINT('Origin',(78.25,48.35,15.775)) ;
#18427=CARTESIAN_POINT('',(80.188427197498,48.35,24.4)) ;
#18428=CARTESIAN_POINT('',(80.188427197498,48.35,25.4)) ;
#18429=CARTESIAN_POINT('',(76.311572802502,48.35,24.4)) ;
#18430=CARTESIAN_POINT('',(76.311572802502,48.35,25.4)) ;
#18431=CARTESIAN_POINT('',(80.45,48.35,24.4)) ;
#18432=CARTESIAN_POINT('Origin',(78.25,47.15,15.775)) ;
#18433=CARTESIAN_POINT('Origin',(82.65,52.3,24.4)) ;
#18434=CARTESIAN_POINT('',(73.85,52.3,24.4)) ;
#18435=CARTESIAN_POINT('Origin',(78.25,52.3,24.4)) ;
#18436=CARTESIAN_POINT('',(76.311572802502,56.25,24.4)) ;
#18437=CARTESIAN_POINT('Origin',(78.25,52.3,24.4)) ;
#18438=CARTESIAN_POINT('',(80.188427197498,56.25,24.4)) ;
#18439=CARTESIAN_POINT('',(80.45,56.25,24.4)) ;
#18440=CARTESIAN_POINT('Origin',(78.25,52.3,24.4)) ;
#18441=CARTESIAN_POINT('Origin',(78.25,56.25,15.775)) ;
#18442=CARTESIAN_POINT('',(80.188427197498,56.25,24.9)) ;
#18443=CARTESIAN_POINT('',(80.188427197498,56.25,25.4)) ;
#18444=CARTESIAN_POINT('',(76.311572802502,56.25,24.9)) ;
#18445=CARTESIAN_POINT('',(76.311572802502,56.25,25.4)) ;
#18446=CARTESIAN_POINT('',(73.25,56.25,24.9)) ;
#18447=CARTESIAN_POINT('',(73.25,56.25,24.9)) ;
#18448=CARTESIAN_POINT('',(73.25,56.25,11.65)) ;
#18449=CARTESIAN_POINT('',(73.25,56.25,11.65)) ;
#18450=CARTESIAN_POINT('',(83.25,56.25,11.65)) ;
#18451=CARTESIAN_POINT('Origin',(78.25,56.25,11.65)) ;
#18452=CARTESIAN_POINT('',(83.25,56.25,24.9)) ;
#18453=CARTESIAN_POINT('',(83.25,56.25,24.9)) ;
#18454=CARTESIAN_POINT('',(73.25,56.25,24.9)) ;
#18455=CARTESIAN_POINT('',(76.2,56.25,11.65)) ;
#18456=CARTESIAN_POINT('Origin',(78.25,56.25,11.65)) ;
#18457=CARTESIAN_POINT('Origin',(78.25,56.25,11.65)) ;
#18458=CARTESIAN_POINT('',(76.2,57.45,11.65)) ;
#18459=CARTESIAN_POINT('Origin',(78.25,57.45,11.65)) ;
#18460=CARTESIAN_POINT('',(76.2,56.25,11.65)) ;
#18461=CARTESIAN_POINT('Origin',(73.25,56.25,11.65)) ;
#18462=CARTESIAN_POINT('',(73.25,57.45,24.9)) ;
#18463=CARTESIAN_POINT('',(73.25,56.25,24.9)) ;
#18464=CARTESIAN_POINT('',(73.25,57.45,11.65)) ;
#18465=CARTESIAN_POINT('',(73.25,57.45,11.65)) ;
#18466=CARTESIAN_POINT('',(73.25,56.25,11.65)) ;
#18467=CARTESIAN_POINT('Origin',(78.25,56.25,11.65)) ;
#18468=CARTESIAN_POINT('',(83.25,57.45,11.65)) ;
#18469=CARTESIAN_POINT('Origin',(78.25,57.45,11.65)) ;
#18470=CARTESIAN_POINT('',(83.25,56.25,11.65)) ;
#18471=CARTESIAN_POINT('Origin',(83.25,56.25,24.9)) ;
#18472=CARTESIAN_POINT('',(83.25,57.45,24.9)) ;
#18473=CARTESIAN_POINT('',(83.25,57.45,24.9)) ;
#18474=CARTESIAN_POINT('',(83.25,56.25,24.9)) ;
#18475=CARTESIAN_POINT('Origin',(73.25,56.25,24.9)) ;
#18476=CARTESIAN_POINT('Origin',(78.25,52.3,24.9)) ;
#18477=CARTESIAN_POINT('',(73.25,57.45,24.9)) ;
#18478=CARTESIAN_POINT('Origin',(78.25,57.45,15.775)) ;
#18479=CARTESIAN_POINT('Origin',(78.25,52.3,25.4)) ;
#18480=CARTESIAN_POINT('',(73.85,52.3,26.4)) ;
#18481=CARTESIAN_POINT('Origin',(78.25,52.3,26.4)) ;
#18482=CARTESIAN_POINT('',(73.85,52.3,25.4)) ;
#18483=CARTESIAN_POINT('Origin',(79.75,52.3,26.)) ;
#18484=CARTESIAN_POINT('',(76.75,52.3,26.)) ;
#18485=CARTESIAN_POINT('Origin',(78.25,52.3,26.)) ;
#18486=CARTESIAN_POINT('Origin',(78.25,52.3,27.)) ;
#18487=CARTESIAN_POINT('',(76.75,52.3,27.6)) ;
#18488=CARTESIAN_POINT('',(76.75,52.3,27.)) ;
#18489=CARTESIAN_POINT('Origin',(78.25,52.3,27.6)) ;
#18490=CARTESIAN_POINT('Origin',(87.25,59.3,26.4)) ;
#18491=CARTESIAN_POINT('',(87.25,59.3,26.4)) ;
#18492=CARTESIAN_POINT('',(69.25,59.3,26.4)) ;
#18493=CARTESIAN_POINT('',(87.25,59.3,26.4)) ;
#18494=CARTESIAN_POINT('',(69.25,59.3,27.6)) ;
#18495=CARTESIAN_POINT('',(69.25,59.3,26.4)) ;
#18496=CARTESIAN_POINT('',(87.25,59.3,27.6)) ;
#18497=CARTESIAN_POINT('',(87.25,59.3,27.6)) ;
#18498=CARTESIAN_POINT('',(87.25,59.3,26.4)) ;
#18499=CARTESIAN_POINT('Origin',(87.25,45.3,26.4)) ;
#18500=CARTESIAN_POINT('',(87.25,45.3,26.4)) ;
#18501=CARTESIAN_POINT('',(87.25,45.3,26.4)) ;
#18502=CARTESIAN_POINT('',(87.25,45.3,27.6)) ;
#18503=CARTESIAN_POINT('',(87.25,45.3,27.6)) ;
#18504=CARTESIAN_POINT('',(87.25,45.3,26.4)) ;
#18505=CARTESIAN_POINT('Origin',(69.25,45.3,26.4)) ;
#18506=CARTESIAN_POINT('',(69.25,45.3,26.4)) ;
#18507=CARTESIAN_POINT('',(69.25,45.3,26.4)) ;
#18508=CARTESIAN_POINT('',(69.25,45.3,27.6)) ;
#18509=CARTESIAN_POINT('',(69.25,45.3,27.6)) ;
#18510=CARTESIAN_POINT('',(69.25,45.3,26.4)) ;
#18511=CARTESIAN_POINT('Origin',(69.25,59.3,26.4)) ;
#18512=CARTESIAN_POINT('',(69.25,59.3,26.4)) ;
#18513=CARTESIAN_POINT('',(69.25,59.3,27.6)) ;
#18514=CARTESIAN_POINT('Origin',(78.25,52.3,27.6)) ;
#18515=CARTESIAN_POINT('Origin',(78.25,52.3,26.4)) ;
#18735=UNCERTAINTY_MEASURE_WITH_UNIT(LENGTH_MEASURE(0.01),#18758,
'DISTANCE_ACCURACY_VALUE',
'Maximum model space distance between geometric entities at asserted c
onnectivities') ;
#18738=UNCERTAINTY_MEASURE_WITH_UNIT(LENGTH_MEASURE(0.01),#18758,
'DISTANCE_ACCURACY_VALUE',
'Maximum model space distance between geometric entities at asserted c
onnectivities') ;
#18754=(
GEOMETRIC_REPRESENTATION_CONTEXT(3)
GLOBAL_UNCERTAINTY_ASSIGNED_CONTEXT((#18735))
GLOBAL_UNIT_ASSIGNED_CONTEXT((#18758,#18760,#18761))
REPRESENTATION_CONTEXT('','3D')
) ;
#18757=(
GEOMETRIC_REPRESENTATION_CONTEXT(3)
GLOBAL_UNCERTAINTY_ASSIGNED_CONTEXT((#18738))
GLOBAL_UNIT_ASSIGNED_CONTEXT((#18758,#18760,#18761))
REPRESENTATION_CONTEXT('','3D')
) ;
#18758=(
LENGTH_UNIT()
NAMED_UNIT(*)
SI_UNIT(.MILLI.,.METRE.)
) ;
#18760=(
NAMED_UNIT(*)
PLANE_ANGLE_UNIT()
SI_UNIT($,.RADIAN.)
) ;
#18761=(
NAMED_UNIT(*)
SI_UNIT($,.STERADIAN.)
SOLID_ANGLE_UNIT()
) ;
#18777=SHAPE_DEFINITION_REPRESENTATION(#18795,#18871) ;
#18795=PRODUCT_DEFINITION_SHAPE('',$,#18890) ;
#18871=SHAPE_REPRESENTATION('',(#10552),#18754) ;
#18874=PRODUCT_DEFINITION_CONTEXT('part definition',#18930,'design') ;
#18890=PRODUCT_DEFINITION('Swivel Caster Yoke 4 in',
'Swivel Caster Yoke 4 in',#18908,#18874) ;
#18908=PRODUCT_DEFINITION_FORMATION('',$,#18947) ;
#18930=APPLICATION_CONTEXT(
'Core Data for Automotive Mechanical Design Process') ;
#18931=PRODUCT_CONTEXT('part definition',#18930,'mechanical') ;
#18947=PRODUCT('Swivel Caster Yoke 4 in','Swivel Caster Yoke 4 in',$,(#18931)) ;
#18965=PRESENTATION_STYLE_ASSIGNMENT((#18983)) ;
#18983=SURFACE_STYLE_USAGE(.BOTH.,#19001) ;
#19001=SURFACE_SIDE_STYLE('',(#19019)) ;
#19019=SURFACE_STYLE_FILL_AREA(#19037) ;
#19037=FILL_AREA_STYLE(
'MAS-253 Metallic Sheet - Swivel Caster Yoke 4 in',(#19055)) ;
#19055=FILL_AREA_STYLE_COLOUR(
'MAS-253 Metallic Sheet - Swivel Caster Yoke 4 in',#19073) ;
#19073=COLOUR_RGB('MAS-253 Metallic Sheet - Swivel Caster Yoke 4 in', 0.40784314, 0.44705882, 0.49803922) ;
ENDSEC;
END-ISO-10303-21;
